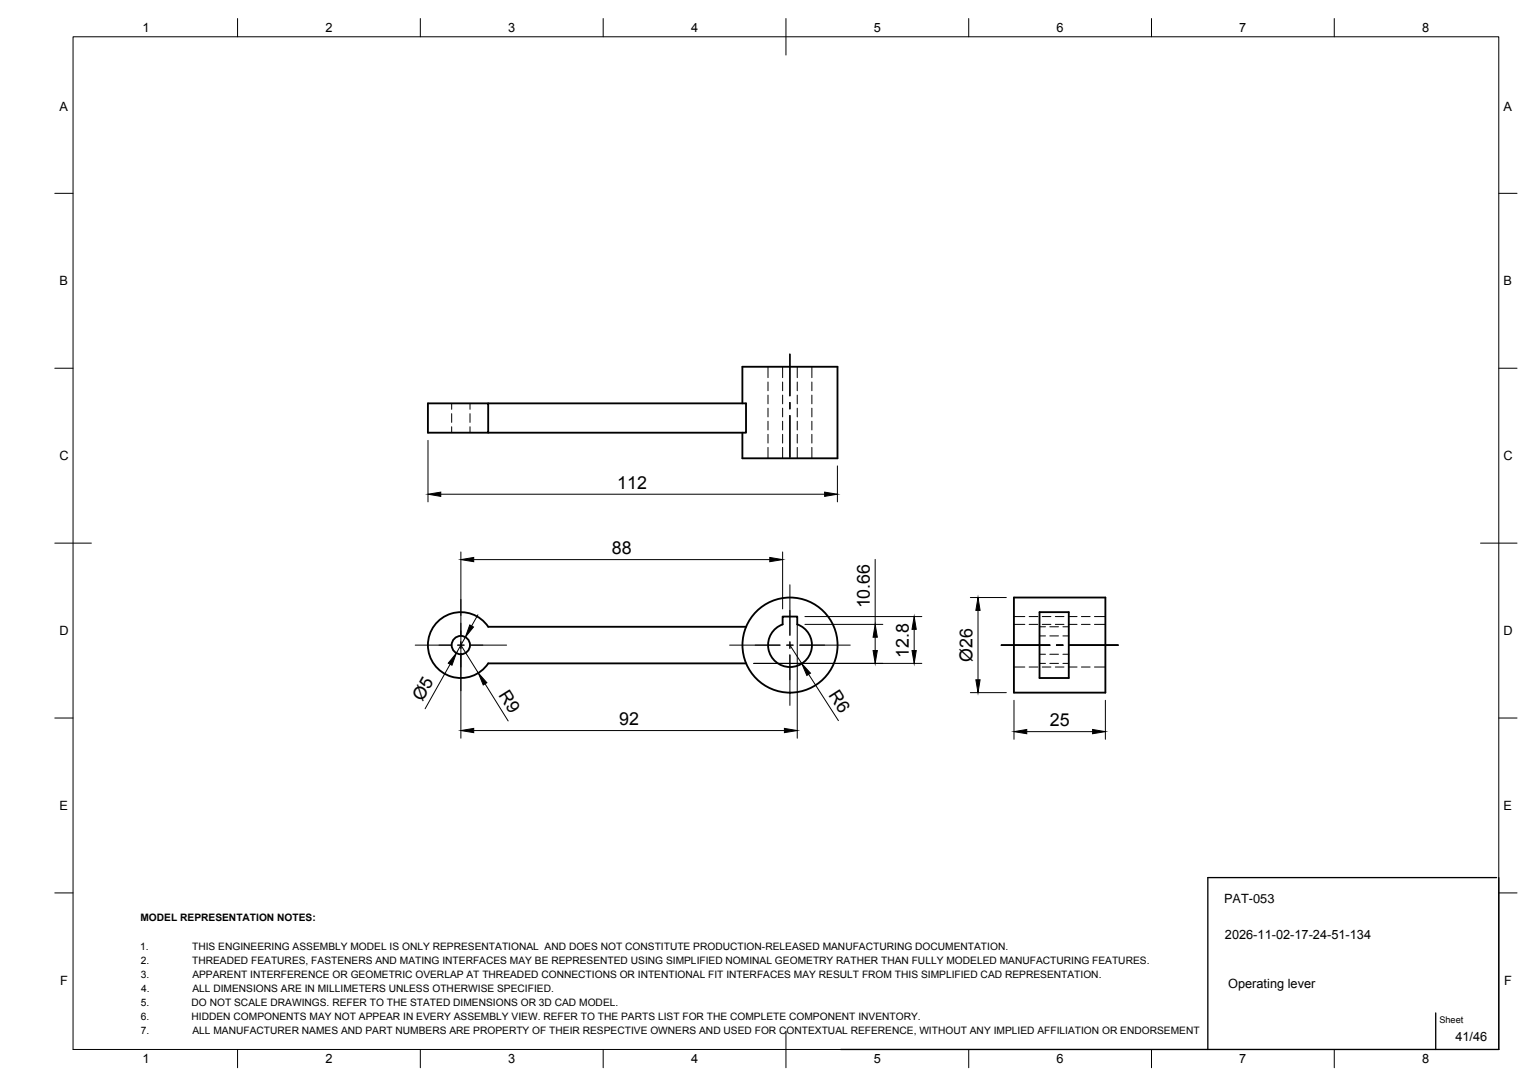
ISO-10303-21;
HEADER;
/* Generated by software containing ST-Developer
 * from STEP Tools, Inc. (www.steptools.com) 
 */

FILE_DESCRIPTION(
/* description */ ('Hand-operated arbor press'),
/* implementation_level */ '2;1');

FILE_NAME(
/* name */ 'Operating lever.step',
/* time_stamp */ '2026-10-28T03:25:25-07:00',
/* author */ (''),
/* organization */ (''),
/* preprocessor_version */ 'ST-DEVELOPER v20.2',
/* originating_system */ 'Autodesk Translation Framework v15.17.0.0',
/* authorisation */ '');

FILE_SCHEMA (('AUTOMOTIVE_DESIGN { 1 0 10303 214 3 1 1 }'));
ENDSEC;

DATA;
#10=MECHANICAL_DESIGN_GEOMETRIC_PRESENTATION_REPRESENTATION('',(#626),#32751);
#535=SHAPE_REPRESENTATION_RELATIONSHIP('SRR','None',#32967,#577);
#577=ADVANCED_BREP_SHAPE_REPRESENTATION('',(#673),#32741);
#626=STYLED_ITEM('',(#33228),#673);
#673=MANIFOLD_SOLID_BREP('Body1',#12525);
#829=FACE_BOUND('',#2654,.T.);
#830=FACE_BOUND('',#2659,.T.);
#831=FACE_BOUND('',#2662,.T.);
#832=FACE_BOUND('',#2664,.T.);
#833=FACE_BOUND('',#2666,.T.);
#1226=PLANE('',#13876);
#1227=PLANE('',#13877);
#1228=PLANE('',#13878);
#1229=PLANE('',#13879);
#1230=PLANE('',#13887);
#1231=PLANE('',#13888);
#1232=PLANE('',#13890);
#1233=PLANE('',#13891);
#1234=PLANE('',#13895);
#1819=FACE_OUTER_BOUND('',#2649,.T.);
#1820=FACE_OUTER_BOUND('',#2650,.T.);
#1821=FACE_OUTER_BOUND('',#2651,.T.);
#1822=FACE_OUTER_BOUND('',#2652,.T.);
#1823=FACE_OUTER_BOUND('',#2653,.T.);
#1824=FACE_OUTER_BOUND('',#2655,.T.);
#1825=FACE_OUTER_BOUND('',#2656,.T.);
#1826=FACE_OUTER_BOUND('',#2657,.T.);
#1827=FACE_OUTER_BOUND('',#2658,.T.);
#1828=FACE_OUTER_BOUND('',#2660,.T.);
#1829=FACE_OUTER_BOUND('',#2661,.T.);
#1830=FACE_OUTER_BOUND('',#2663,.T.);
#1831=FACE_OUTER_BOUND('',#2665,.T.);
#2649=EDGE_LOOP('',(#10884,#10885,#10886,#10887));
#2650=EDGE_LOOP('',(#10888,#10889,#10890,#10891));
#2651=EDGE_LOOP('',(#10892,#10893,#10894,#10895));
#2652=EDGE_LOOP('',(#10896,#10897,#10898,#10899));
#2653=EDGE_LOOP('',(#10900));
#2654=EDGE_LOOP('',(#10901,#10902,#10903,#10904));
#2655=EDGE_LOOP('',(#10905,#10906,#10907,#10908));
#2656=EDGE_LOOP('',(#10909,#10910,#10911,#10912));
#2657=EDGE_LOOP('',(#10913,#10914,#10915,#10916));
#2658=EDGE_LOOP('',(#10917,#10918,#10919,#10920));
#2659=EDGE_LOOP('',(#10921));
#2660=EDGE_LOOP('',(#10922,#10923,#10924,#10925));
#2661=EDGE_LOOP('',(#10926,#10927,#10928,#10929));
#2662=EDGE_LOOP('',(#10930));
#2663=EDGE_LOOP('',(#10931,#10932,#10933,#10934));
#2664=EDGE_LOOP('',(#10935,#10936,#10937,#10938));
#2665=EDGE_LOOP('',(#10939));
#2666=EDGE_LOOP('',(#10940,#10941,#10942,#10943));
#3786=LINE('',#20717,#4957);
#3787=LINE('',#20722,#4958);
#3788=LINE('',#20724,#4959);
#3789=LINE('',#20726,#4960);
#3790=LINE('',#20727,#4961);
#3791=LINE('',#20730,#4962);
#3792=LINE('',#20732,#4963);
#3793=LINE('',#20733,#4964);
#3794=LINE('',#20736,#4965);
#3795=LINE('',#20738,#4966);
#3796=LINE('',#20739,#4967);
#3797=LINE('',#20749,#4968);
#3798=LINE('',#20753,#4969);
#3799=LINE('',#20757,#4970);
#3800=LINE('',#20759,#4971);
#3801=LINE('',#20760,#4972);
#3802=LINE('',#20763,#4973);
#3803=LINE('',#20767,#4974);
#3804=LINE('',#20768,#4975);
#3805=LINE('',#20773,#4976);
#4957=VECTOR('',#16869,0.25);
#4958=VECTOR('',#16874,1.);
#4959=VECTOR('',#16875,1.);
#4960=VECTOR('',#16876,1.);
#4961=VECTOR('',#16877,1.);
#4962=VECTOR('',#16880,1.);
#4963=VECTOR('',#16881,1.);
#4964=VECTOR('',#16882,1.);
#4965=VECTOR('',#16885,1.);
#4966=VECTOR('',#16886,1.);
#4967=VECTOR('',#16887,1.);
#4968=VECTOR('',#16900,1.);
#4969=VECTOR('',#16903,1.);
#4970=VECTOR('',#16908,1.);
#4971=VECTOR('',#16909,1.);
#4972=VECTOR('',#16910,1.);
#4973=VECTOR('',#16913,1.);
#4974=VECTOR('',#16918,1.);
#4975=VECTOR('',#16919,1.);
#4976=VECTOR('',#16926,1.3);
#5466=CIRCLE('',#13874,0.25);
#5467=CIRCLE('',#13875,0.25);
#5468=CIRCLE('',#13880,1.3);
#5469=CIRCLE('',#13881,0.6);
#5470=CIRCLE('',#13883,0.6);
#5471=CIRCLE('',#13885,0.9);
#5472=CIRCLE('',#13886,0.9);
#5473=CIRCLE('',#13889,1.3);
#5474=CIRCLE('',#13892,1.3);
#5475=CIRCLE('',#13894,1.3);
#6415=VERTEX_POINT('',#20714);
#6416=VERTEX_POINT('',#20716);
#6417=VERTEX_POINT('',#20720);
#6418=VERTEX_POINT('',#20721);
#6419=VERTEX_POINT('',#20723);
#6420=VERTEX_POINT('',#20725);
#6421=VERTEX_POINT('',#20729);
#6422=VERTEX_POINT('',#20731);
#6423=VERTEX_POINT('',#20735);
#6424=VERTEX_POINT('',#20737);
#6425=VERTEX_POINT('',#20741);
#6426=VERTEX_POINT('',#20747);
#6427=VERTEX_POINT('',#20748);
#6428=VERTEX_POINT('',#20750);
#6429=VERTEX_POINT('',#20752);
#6430=VERTEX_POINT('',#20756);
#6431=VERTEX_POINT('',#20758);
#6432=VERTEX_POINT('',#20762);
#6433=VERTEX_POINT('',#20766);
#6434=VERTEX_POINT('',#20772);
#7945=EDGE_CURVE('',#6415,#6415,#5466,.T.);
#7946=EDGE_CURVE('',#6415,#6416,#3786,.T.);
#7947=EDGE_CURVE('',#6416,#6416,#5467,.T.);
#7948=EDGE_CURVE('',#6417,#6418,#3787,.T.);
#7949=EDGE_CURVE('',#6417,#6419,#3788,.T.);
#7950=EDGE_CURVE('',#6420,#6419,#3789,.T.);
#7951=EDGE_CURVE('',#6418,#6420,#3790,.T.);
#7952=EDGE_CURVE('',#6421,#6417,#3791,.T.);
#7953=EDGE_CURVE('',#6421,#6422,#3792,.T.);
#7954=EDGE_CURVE('',#6419,#6422,#3793,.T.);
#7955=EDGE_CURVE('',#6423,#6421,#3794,.T.);
#7956=EDGE_CURVE('',#6424,#6423,#3795,.T.);
#7957=EDGE_CURVE('',#6422,#6424,#3796,.T.);
#7958=EDGE_CURVE('',#6425,#6425,#5468,.T.);
#7959=EDGE_CURVE('',#6424,#6420,#5469,.T.);
#7960=EDGE_CURVE('',#6423,#6418,#5470,.T.);
#7961=EDGE_CURVE('',#6426,#6427,#3797,.T.);
#7962=EDGE_CURVE('',#6428,#6426,#5471,.T.);
#7963=EDGE_CURVE('',#6429,#6428,#3798,.T.);
#7964=EDGE_CURVE('',#6429,#6427,#5472,.T.);
#7965=EDGE_CURVE('',#6430,#6427,#3799,.T.);
#7966=EDGE_CURVE('',#6431,#6430,#3800,.T.);
#7967=EDGE_CURVE('',#6426,#6431,#3801,.T.);
#7968=EDGE_CURVE('',#6429,#6432,#3802,.T.);
#7969=EDGE_CURVE('',#6430,#6432,#5473,.T.);
#7970=EDGE_CURVE('',#6433,#6428,#3803,.T.);
#7971=EDGE_CURVE('',#6432,#6433,#3804,.T.);
#7972=EDGE_CURVE('',#6433,#6431,#5474,.T.);
#7973=EDGE_CURVE('',#6425,#6434,#3805,.T.);
#7974=EDGE_CURVE('',#6434,#6434,#5475,.T.);
#10884=ORIENTED_EDGE('',*,*,#7945,.F.);
#10885=ORIENTED_EDGE('',*,*,#7946,.T.);
#10886=ORIENTED_EDGE('',*,*,#7947,.F.);
#10887=ORIENTED_EDGE('',*,*,#7946,.F.);
#10888=ORIENTED_EDGE('',*,*,#7948,.F.);
#10889=ORIENTED_EDGE('',*,*,#7949,.T.);
#10890=ORIENTED_EDGE('',*,*,#7950,.F.);
#10891=ORIENTED_EDGE('',*,*,#7951,.F.);
#10892=ORIENTED_EDGE('',*,*,#7952,.F.);
#10893=ORIENTED_EDGE('',*,*,#7953,.T.);
#10894=ORIENTED_EDGE('',*,*,#7954,.F.);
#10895=ORIENTED_EDGE('',*,*,#7949,.F.);
#10896=ORIENTED_EDGE('',*,*,#7955,.F.);
#10897=ORIENTED_EDGE('',*,*,#7956,.F.);
#10898=ORIENTED_EDGE('',*,*,#7957,.F.);
#10899=ORIENTED_EDGE('',*,*,#7953,.F.);
#10900=ORIENTED_EDGE('',*,*,#7958,.T.);
#10901=ORIENTED_EDGE('',*,*,#7950,.T.);
#10902=ORIENTED_EDGE('',*,*,#7954,.T.);
#10903=ORIENTED_EDGE('',*,*,#7957,.T.);
#10904=ORIENTED_EDGE('',*,*,#7959,.T.);
#10905=ORIENTED_EDGE('',*,*,#7951,.T.);
#10906=ORIENTED_EDGE('',*,*,#7959,.F.);
#10907=ORIENTED_EDGE('',*,*,#7956,.T.);
#10908=ORIENTED_EDGE('',*,*,#7960,.T.);
#10909=ORIENTED_EDGE('',*,*,#7961,.F.);
#10910=ORIENTED_EDGE('',*,*,#7962,.F.);
#10911=ORIENTED_EDGE('',*,*,#7963,.F.);
#10912=ORIENTED_EDGE('',*,*,#7964,.T.);
#10913=ORIENTED_EDGE('',*,*,#7961,.T.);
#10914=ORIENTED_EDGE('',*,*,#7965,.F.);
#10915=ORIENTED_EDGE('',*,*,#7966,.F.);
#10916=ORIENTED_EDGE('',*,*,#7967,.F.);
#10917=ORIENTED_EDGE('',*,*,#7964,.F.);
#10918=ORIENTED_EDGE('',*,*,#7968,.T.);
#10919=ORIENTED_EDGE('',*,*,#7969,.F.);
#10920=ORIENTED_EDGE('',*,*,#7965,.T.);
#10921=ORIENTED_EDGE('',*,*,#7945,.T.);
#10922=ORIENTED_EDGE('',*,*,#7963,.T.);
#10923=ORIENTED_EDGE('',*,*,#7970,.F.);
#10924=ORIENTED_EDGE('',*,*,#7971,.F.);
#10925=ORIENTED_EDGE('',*,*,#7968,.F.);
#10926=ORIENTED_EDGE('',*,*,#7967,.T.);
#10927=ORIENTED_EDGE('',*,*,#7972,.F.);
#10928=ORIENTED_EDGE('',*,*,#7970,.T.);
#10929=ORIENTED_EDGE('',*,*,#7962,.T.);
#10930=ORIENTED_EDGE('',*,*,#7947,.T.);
#10931=ORIENTED_EDGE('',*,*,#7958,.F.);
#10932=ORIENTED_EDGE('',*,*,#7973,.T.);
#10933=ORIENTED_EDGE('',*,*,#7974,.T.);
#10934=ORIENTED_EDGE('',*,*,#7973,.F.);
#10935=ORIENTED_EDGE('',*,*,#7966,.T.);
#10936=ORIENTED_EDGE('',*,*,#7969,.T.);
#10937=ORIENTED_EDGE('',*,*,#7971,.T.);
#10938=ORIENTED_EDGE('',*,*,#7972,.T.);
#10939=ORIENTED_EDGE('',*,*,#7974,.F.);
#10940=ORIENTED_EDGE('',*,*,#7948,.T.);
#10941=ORIENTED_EDGE('',*,*,#7960,.F.);
#10942=ORIENTED_EDGE('',*,*,#7955,.T.);
#10943=ORIENTED_EDGE('',*,*,#7952,.T.);
#11762=CYLINDRICAL_SURFACE('',#13873,0.25);
#11763=CYLINDRICAL_SURFACE('',#13882,0.6);
#11764=CYLINDRICAL_SURFACE('',#13884,0.9);
#11765=CYLINDRICAL_SURFACE('',#13893,1.3);
#12328=ADVANCED_FACE('',(#1819),#11762,.F.);
#12329=ADVANCED_FACE('',(#1820),#1226,.F.);
#12330=ADVANCED_FACE('',(#1821),#1227,.F.);
#12331=ADVANCED_FACE('',(#1822),#1228,.F.);
#12332=ADVANCED_FACE('',(#1823,#829),#1229,.T.);
#12333=ADVANCED_FACE('',(#1824),#11763,.F.);
#12334=ADVANCED_FACE('',(#1825),#11764,.T.);
#12335=ADVANCED_FACE('',(#1826),#1230,.T.);
#12336=ADVANCED_FACE('',(#1827,#830),#1231,.F.);
#12337=ADVANCED_FACE('',(#1828),#1232,.T.);
#12338=ADVANCED_FACE('',(#1829,#831),#1233,.T.);
#12339=ADVANCED_FACE('',(#1830,#832),#11765,.T.);
#12340=ADVANCED_FACE('',(#1831,#833),#1234,.F.);
#12525=CLOSED_SHELL('',(#12328,#12329,#12330,#12331,#12332,#12333,#12334,
#12335,#12336,#12337,#12338,#12339,#12340));
#13872=AXIS2_PLACEMENT_3D('',#20712,#16863,#16864);
#13873=AXIS2_PLACEMENT_3D('',#20713,#16865,#16866);
#13874=AXIS2_PLACEMENT_3D('',#20715,#16867,#16868);
#13875=AXIS2_PLACEMENT_3D('',#20718,#16870,#16871);
#13876=AXIS2_PLACEMENT_3D('',#20719,#16872,#16873);
#13877=AXIS2_PLACEMENT_3D('',#20728,#16878,#16879);
#13878=AXIS2_PLACEMENT_3D('',#20734,#16883,#16884);
#13879=AXIS2_PLACEMENT_3D('',#20740,#16888,#16889);
#13880=AXIS2_PLACEMENT_3D('',#20742,#16890,#16891);
#13881=AXIS2_PLACEMENT_3D('',#20743,#16892,#16893);
#13882=AXIS2_PLACEMENT_3D('',#20744,#16894,#16895);
#13883=AXIS2_PLACEMENT_3D('',#20745,#16896,#16897);
#13884=AXIS2_PLACEMENT_3D('',#20746,#16898,#16899);
#13885=AXIS2_PLACEMENT_3D('',#20751,#16901,#16902);
#13886=AXIS2_PLACEMENT_3D('',#20754,#16904,#16905);
#13887=AXIS2_PLACEMENT_3D('',#20755,#16906,#16907);
#13888=AXIS2_PLACEMENT_3D('',#20761,#16911,#16912);
#13889=AXIS2_PLACEMENT_3D('',#20764,#16914,#16915);
#13890=AXIS2_PLACEMENT_3D('',#20765,#16916,#16917);
#13891=AXIS2_PLACEMENT_3D('',#20769,#16920,#16921);
#13892=AXIS2_PLACEMENT_3D('',#20770,#16922,#16923);
#13893=AXIS2_PLACEMENT_3D('',#20771,#16924,#16925);
#13894=AXIS2_PLACEMENT_3D('',#20774,#16927,#16928);
#13895=AXIS2_PLACEMENT_3D('',#20775,#16929,#16930);
#16863=DIRECTION('axis',(0.,0.,1.));
#16864=DIRECTION('refdir',(1.,0.,0.));
#16865=DIRECTION('center_axis',(0.,1.,0.));
#16866=DIRECTION('ref_axis',(1.,0.,0.));
#16867=DIRECTION('center_axis',(0.,1.,0.));
#16868=DIRECTION('ref_axis',(1.,0.,0.));
#16869=DIRECTION('',(0.,1.,0.));
#16870=DIRECTION('center_axis',(0.,-1.,0.));
#16871=DIRECTION('ref_axis',(1.,0.,0.));
#16872=DIRECTION('center_axis',(0.,0.,-1.));
#16873=DIRECTION('ref_axis',(-1.,0.,0.));
#16874=DIRECTION('',(-1.,0.,0.));
#16875=DIRECTION('',(0.,1.,0.));
#16876=DIRECTION('',(1.,0.,0.));
#16877=DIRECTION('',(0.,1.,0.));
#16878=DIRECTION('center_axis',(1.,0.,0.));
#16879=DIRECTION('ref_axis',(0.,0.,-1.));
#16880=DIRECTION('',(0.,0.,-1.));
#16881=DIRECTION('',(0.,1.,0.));
#16882=DIRECTION('',(0.,0.,1.));
#16883=DIRECTION('center_axis',(0.,0.,1.));
#16884=DIRECTION('ref_axis',(1.,0.,0.));
#16885=DIRECTION('',(1.,0.,0.));
#16886=DIRECTION('',(0.,-1.,0.));
#16887=DIRECTION('',(-1.,0.,0.));
#16888=DIRECTION('center_axis',(0.,1.,0.));
#16889=DIRECTION('ref_axis',(1.,0.,0.));
#16890=DIRECTION('center_axis',(0.,1.,0.));
#16891=DIRECTION('ref_axis',(1.,0.,0.));
#16892=DIRECTION('center_axis',(0.,-1.,0.));
#16893=DIRECTION('ref_axis',(1.,0.,0.));
#16894=DIRECTION('center_axis',(0.,1.,0.));
#16895=DIRECTION('ref_axis',(-1.,0.,-1.22464679914735E-16));
#16896=DIRECTION('center_axis',(0.,-1.,0.));
#16897=DIRECTION('ref_axis',(1.,0.,0.));
#16898=DIRECTION('center_axis',(0.,1.,0.));
#16899=DIRECTION('ref_axis',(6.12323399573677E-17,0.,1.));
#16900=DIRECTION('',(0.,-1.,0.));
#16901=DIRECTION('center_axis',(0.,1.,0.));
#16902=DIRECTION('ref_axis',(1.,0.,0.));
#16903=DIRECTION('',(0.,1.,0.));
#16904=DIRECTION('center_axis',(0.,1.,0.));
#16905=DIRECTION('ref_axis',(1.,0.,0.));
#16906=DIRECTION('center_axis',(1.,0.,0.));
#16907=DIRECTION('ref_axis',(0.,0.,-1.));
#16908=DIRECTION('',(0.,0.,1.));
#16909=DIRECTION('',(0.,-1.,0.));
#16910=DIRECTION('',(0.,0.,-1.));
#16911=DIRECTION('center_axis',(0.,1.,0.));
#16912=DIRECTION('ref_axis',(1.,0.,0.));
#16913=DIRECTION('',(0.,0.,-1.));
#16914=DIRECTION('center_axis',(0.,-1.,0.));
#16915=DIRECTION('ref_axis',(1.,0.,0.));
#16916=DIRECTION('center_axis',(-1.,0.,0.));
#16917=DIRECTION('ref_axis',(0.,0.,1.));
#16918=DIRECTION('',(0.,0.,1.));
#16919=DIRECTION('',(0.,1.,0.));
#16920=DIRECTION('center_axis',(0.,1.,0.));
#16921=DIRECTION('ref_axis',(0.,0.,1.));
#16922=DIRECTION('center_axis',(0.,1.,0.));
#16923=DIRECTION('ref_axis',(1.,0.,0.));
#16924=DIRECTION('center_axis',(0.,1.,0.));
#16925=DIRECTION('ref_axis',(1.,0.,0.));
#16926=DIRECTION('',(0.,-1.,0.));
#16927=DIRECTION('center_axis',(0.,1.,0.));
#16928=DIRECTION('ref_axis',(1.,0.,0.));
#16929=DIRECTION('center_axis',(0.,1.,0.));
#16930=DIRECTION('ref_axis',(1.,0.,0.));
#20712=CARTESIAN_POINT('',(0.,0.,0.));
#20713=CARTESIAN_POINT('Origin',(-3.25,5.9,29.));
#20714=CARTESIAN_POINT('',(-3.5,6.,29.));
#20715=CARTESIAN_POINT('Origin',(-3.25,6.,29.));
#20716=CARTESIAN_POINT('',(-3.5,6.8,29.));
#20717=CARTESIAN_POINT('',(-3.5,5.9,29.));
#20718=CARTESIAN_POINT('Origin',(-3.25,6.8,29.));
#20719=CARTESIAN_POINT('Origin',(-2.47,4.9,19.8));
#20720=CARTESIAN_POINT('',(-2.47,5.,19.8));
#20721=CARTESIAN_POINT('',(-2.68431457505076,5.,19.8));
#20722=CARTESIAN_POINT('',(-2.86,5.,19.8));
#20723=CARTESIAN_POINT('',(-2.47,7.5,19.8));
#20724=CARTESIAN_POINT('',(-2.47,4.9,19.8));
#20725=CARTESIAN_POINT('',(-2.68431457505076,7.5,19.8));
#20726=CARTESIAN_POINT('',(-2.86,7.5,19.8));
#20727=CARTESIAN_POINT('',(-2.68431457505076,5.,19.8));
#20728=CARTESIAN_POINT('Origin',(-2.47,4.9,20.2));
#20729=CARTESIAN_POINT('',(-2.47,5.,20.2));
#20730=CARTESIAN_POINT('',(-2.47,5.,20.1));
#20731=CARTESIAN_POINT('',(-2.47,7.5,20.2));
#20732=CARTESIAN_POINT('',(-2.47,4.9,20.2));
#20733=CARTESIAN_POINT('',(-2.47,7.5,20.1));
#20734=CARTESIAN_POINT('Origin',(-2.9,4.9,20.2));
#20735=CARTESIAN_POINT('',(-2.68431457505076,5.,20.2));
#20736=CARTESIAN_POINT('',(-3.075,5.,20.2));
#20737=CARTESIAN_POINT('',(-2.68431457505076,7.5,20.2));
#20738=CARTESIAN_POINT('',(-2.68431457505076,5.,20.2));
#20739=CARTESIAN_POINT('',(-3.075,7.5,20.2));
#20740=CARTESIAN_POINT('Origin',(-3.25,7.5,20.));
#20741=CARTESIAN_POINT('',(-4.55,7.5,20.));
#20742=CARTESIAN_POINT('Origin',(-3.25,7.5,20.));
#20743=CARTESIAN_POINT('Origin',(-3.25,7.5,20.));
#20744=CARTESIAN_POINT('Origin',(-3.25,5.,20.));
#20745=CARTESIAN_POINT('Origin',(-3.25,5.,20.));
#20746=CARTESIAN_POINT('Origin',(-3.25,6.,29.));
#20747=CARTESIAN_POINT('',(-2.75,6.8,28.2516685226452));
#20748=CARTESIAN_POINT('',(-2.75,6.,28.2516685226452));
#20749=CARTESIAN_POINT('',(-2.75,6.,28.2516685226452));
#20750=CARTESIAN_POINT('',(-3.75,6.8,28.2516685226452));
#20751=CARTESIAN_POINT('Origin',(-3.25,6.8,29.));
#20752=CARTESIAN_POINT('',(-3.75,6.,28.2516685226452));
#20753=CARTESIAN_POINT('',(-3.75,6.,28.2516685226452));
#20754=CARTESIAN_POINT('Origin',(-3.25,6.,29.));
#20755=CARTESIAN_POINT('Origin',(-2.75,6.,29.));
#20756=CARTESIAN_POINT('',(-2.75,6.,21.2));
#20757=CARTESIAN_POINT('',(-2.75,6.,20.));
#20758=CARTESIAN_POINT('',(-2.75,6.8,21.2));
#20759=CARTESIAN_POINT('',(-2.75,5.,21.2));
#20760=CARTESIAN_POINT('',(-2.75,6.8,20.));
#20761=CARTESIAN_POINT('Origin',(-3.25,6.,24.5));
#20762=CARTESIAN_POINT('',(-3.75,6.,21.2));
#20763=CARTESIAN_POINT('',(-3.75,6.,29.));
#20764=CARTESIAN_POINT('Origin',(-3.25,6.,20.));
#20765=CARTESIAN_POINT('Origin',(-3.75,6.,20.));
#20766=CARTESIAN_POINT('',(-3.75,6.8,21.2));
#20767=CARTESIAN_POINT('',(-3.75,6.8,29.));
#20768=CARTESIAN_POINT('',(-3.75,5.,21.2));
#20769=CARTESIAN_POINT('Origin',(-3.25,6.8,24.5));
#20770=CARTESIAN_POINT('Origin',(-3.25,6.8,20.));
#20771=CARTESIAN_POINT('Origin',(-3.25,5.,20.));
#20772=CARTESIAN_POINT('',(-4.55,5.,20.));
#20773=CARTESIAN_POINT('',(-4.55,5.,20.));
#20774=CARTESIAN_POINT('Origin',(-3.25,5.,20.));
#20775=CARTESIAN_POINT('Origin',(-3.25,5.,20.));
#32692=UNCERTAINTY_MEASURE_WITH_UNIT(LENGTH_MEASURE(0.001),#32752,
'DISTANCE_ACCURACY_VALUE',
'Maximum model space distance between geometric entities at asserted c
onnectivities');
#32702=UNCERTAINTY_MEASURE_WITH_UNIT(LENGTH_MEASURE(0.001),#32752,
'DISTANCE_ACCURACY_VALUE',
'Maximum model space distance between geometric entities at asserted c
onnectivities');
#32741=(
GEOMETRIC_REPRESENTATION_CONTEXT(3)
GLOBAL_UNCERTAINTY_ASSIGNED_CONTEXT((#32692))
GLOBAL_UNIT_ASSIGNED_CONTEXT((#32752,#32754,#32755))
REPRESENTATION_CONTEXT('','3D')
);
#32751=(
GEOMETRIC_REPRESENTATION_CONTEXT(3)
GLOBAL_UNCERTAINTY_ASSIGNED_CONTEXT((#32702))
GLOBAL_UNIT_ASSIGNED_CONTEXT((#32752,#32754,#32755))
REPRESENTATION_CONTEXT('','3D')
);
#32752=(
LENGTH_UNIT()
NAMED_UNIT(*)
SI_UNIT(.CENTI.,.METRE.)
);
#32754=(
NAMED_UNIT(*)
PLANE_ANGLE_UNIT()
SI_UNIT($,.RADIAN.)
);
#32755=(
NAMED_UNIT(*)
SI_UNIT($,.STERADIAN.)
SOLID_ANGLE_UNIT()
);
#32794=SHAPE_DEFINITION_REPRESENTATION(#32851,#32967);
#32851=PRODUCT_DEFINITION_SHAPE('',$,#33016);
#32967=SHAPE_REPRESENTATION('',(#13872),#32741);
#32977=PRODUCT_DEFINITION_CONTEXT('part definition',#33123,'design');
#33016=PRODUCT_DEFINITION('Operating lever','Operating lever',#33064,#32977);
#33064=PRODUCT_DEFINITION_FORMATION('',$,#33163);
#33123=APPLICATION_CONTEXT(
'Core Data for Automotive Mechanical Design Process');
#33124=PRODUCT_CONTEXT('part definition',#33123,'mechanical');
#33163=PRODUCT('Operating lever','Operating lever','Operating lever',(#33124));
#33222=COLOUR_RGB('Light Blue',0.38,0.62,0.78);
#33223=FILL_AREA_STYLE_COLOUR('',#33222);
#33224=FILL_AREA_STYLE('',(#33223));
#33225=SURFACE_STYLE_FILL_AREA(#33224);
#33226=SURFACE_SIDE_STYLE('',(#33225));
#33227=SURFACE_STYLE_USAGE(.BOTH.,#33226);
#33228=PRESENTATION_STYLE_ASSIGNMENT((#33227));
ENDSEC;
END-ISO-10303-21;
